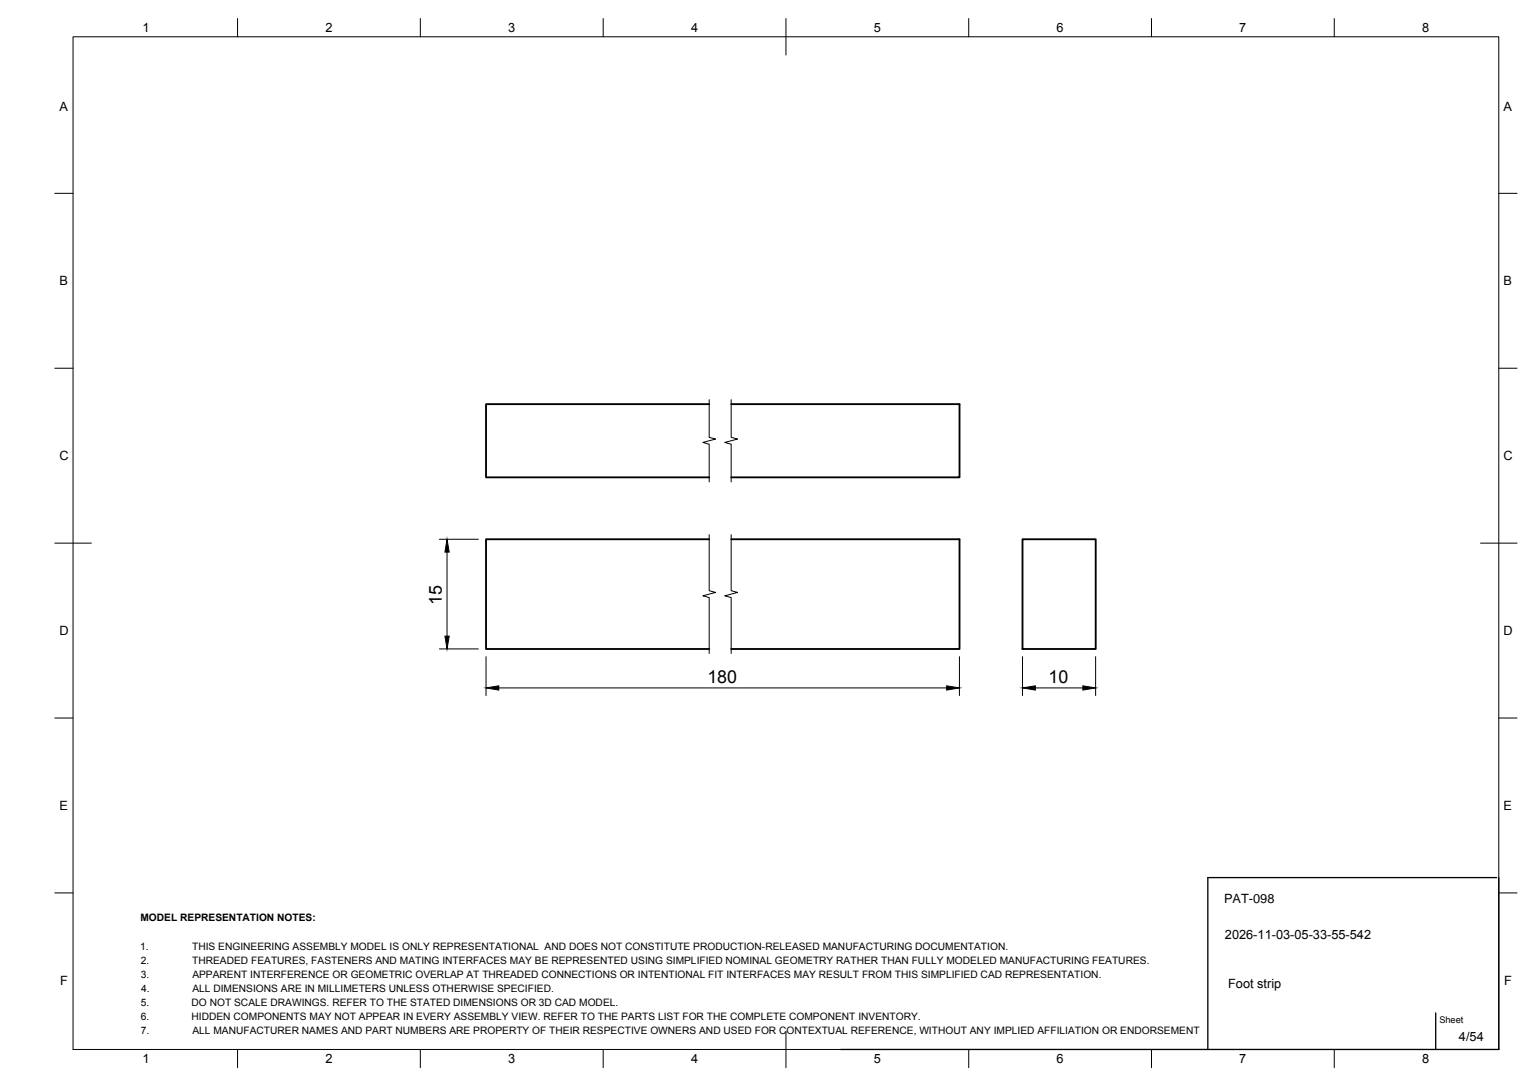
ISO-10303-21;
HEADER;
/* Generated by software containing ST-Developer
 * from STEP Tools, Inc. (www.steptools.com) 
 */

FILE_DESCRIPTION(
/* description */ ('Spring compression tester'),
/* implementation_level */ '2;1');

FILE_NAME(
/* name */ 'Foot strip.step',
/* time_stamp */ '2026-10-28T03:24:11-07:00',
/* author */ (''),
/* organization */ (''),
/* preprocessor_version */ 'ST-DEVELOPER v20.2',
/* originating_system */ 'Autodesk Translation Framework v15.17.0.0',
/* authorisation */ '');

FILE_SCHEMA (('AUTOMOTIVE_DESIGN { 1 0 10303 214 3 1 1 }'));
ENDSEC;

DATA;
#10=MECHANICAL_DESIGN_GEOMETRIC_PRESENTATION_REPRESENTATION('',(#1105),#43521);
#985=SHAPE_REPRESENTATION_RELATIONSHIP('SRR','None',#43797,#1045);
#1045=ADVANCED_BREP_SHAPE_REPRESENTATION('',(#1180),#43457);
#1105=STYLED_ITEM('',(#44188),#1180);
#1180=MANIFOLD_SOLID_BREP('Body1',#18542);
#1603=PLANE('',#19362);
#1604=PLANE('',#19363);
#1605=PLANE('',#19364);
#1606=PLANE('',#19365);
#1607=PLANE('',#19366);
#1608=PLANE('',#19367);
#2204=FACE_OUTER_BOUND('',#3287,.T.);
#2205=FACE_OUTER_BOUND('',#3288,.T.);
#2206=FACE_OUTER_BOUND('',#3289,.T.);
#2207=FACE_OUTER_BOUND('',#3290,.T.);
#2208=FACE_OUTER_BOUND('',#3291,.T.);
#2209=FACE_OUTER_BOUND('',#3292,.T.);
#3287=EDGE_LOOP('',(#12385,#12386,#12387,#12388));
#3288=EDGE_LOOP('',(#12389,#12390,#12391,#12392));
#3289=EDGE_LOOP('',(#12393,#12394,#12395,#12396));
#3290=EDGE_LOOP('',(#12397,#12398,#12399,#12400));
#3291=EDGE_LOOP('',(#12401,#12402,#12403,#12404));
#3292=EDGE_LOOP('',(#12405,#12406,#12407,#12408));
#4650=LINE('',#26633,#6082);
#4651=LINE('',#26635,#6083);
#4652=LINE('',#26637,#6084);
#4653=LINE('',#26638,#6085);
#4654=LINE('',#26641,#6086);
#4655=LINE('',#26643,#6087);
#4656=LINE('',#26644,#6088);
#4657=LINE('',#26647,#6089);
#4658=LINE('',#26649,#6090);
#4659=LINE('',#26650,#6091);
#4660=LINE('',#26652,#6092);
#4661=LINE('',#26653,#6093);
#6082=VECTOR('',#21398,1.);
#6083=VECTOR('',#21399,1.);
#6084=VECTOR('',#21400,1.);
#6085=VECTOR('',#21401,1.);
#6086=VECTOR('',#21404,1.);
#6087=VECTOR('',#21405,1.);
#6088=VECTOR('',#21406,1.);
#6089=VECTOR('',#21409,1.);
#6090=VECTOR('',#21410,1.);
#6091=VECTOR('',#21411,1.);
#6092=VECTOR('',#21414,1.);
#6093=VECTOR('',#21415,1.);
#8192=VERTEX_POINT('',#26631);
#8193=VERTEX_POINT('',#26632);
#8194=VERTEX_POINT('',#26634);
#8195=VERTEX_POINT('',#26636);
#8196=VERTEX_POINT('',#26640);
#8197=VERTEX_POINT('',#26642);
#8198=VERTEX_POINT('',#26646);
#8199=VERTEX_POINT('',#26648);
#9857=EDGE_CURVE('',#8192,#8193,#4650,.T.);
#9858=EDGE_CURVE('',#8193,#8194,#4651,.T.);
#9859=EDGE_CURVE('',#8195,#8194,#4652,.T.);
#9860=EDGE_CURVE('',#8192,#8195,#4653,.T.);
#9861=EDGE_CURVE('',#8196,#8192,#4654,.T.);
#9862=EDGE_CURVE('',#8197,#8195,#4655,.T.);
#9863=EDGE_CURVE('',#8196,#8197,#4656,.T.);
#9864=EDGE_CURVE('',#8198,#8196,#4657,.T.);
#9865=EDGE_CURVE('',#8199,#8197,#4658,.T.);
#9866=EDGE_CURVE('',#8198,#8199,#4659,.T.);
#9867=EDGE_CURVE('',#8193,#8198,#4660,.T.);
#9868=EDGE_CURVE('',#8194,#8199,#4661,.T.);
#12385=ORIENTED_EDGE('',*,*,#9857,.T.);
#12386=ORIENTED_EDGE('',*,*,#9858,.T.);
#12387=ORIENTED_EDGE('',*,*,#9859,.F.);
#12388=ORIENTED_EDGE('',*,*,#9860,.F.);
#12389=ORIENTED_EDGE('',*,*,#9861,.T.);
#12390=ORIENTED_EDGE('',*,*,#9860,.T.);
#12391=ORIENTED_EDGE('',*,*,#9862,.F.);
#12392=ORIENTED_EDGE('',*,*,#9863,.F.);
#12393=ORIENTED_EDGE('',*,*,#9864,.T.);
#12394=ORIENTED_EDGE('',*,*,#9863,.T.);
#12395=ORIENTED_EDGE('',*,*,#9865,.F.);
#12396=ORIENTED_EDGE('',*,*,#9866,.F.);
#12397=ORIENTED_EDGE('',*,*,#9867,.T.);
#12398=ORIENTED_EDGE('',*,*,#9866,.T.);
#12399=ORIENTED_EDGE('',*,*,#9868,.F.);
#12400=ORIENTED_EDGE('',*,*,#9858,.F.);
#12401=ORIENTED_EDGE('',*,*,#9868,.T.);
#12402=ORIENTED_EDGE('',*,*,#9865,.T.);
#12403=ORIENTED_EDGE('',*,*,#9862,.T.);
#12404=ORIENTED_EDGE('',*,*,#9859,.T.);
#12405=ORIENTED_EDGE('',*,*,#9867,.F.);
#12406=ORIENTED_EDGE('',*,*,#9857,.F.);
#12407=ORIENTED_EDGE('',*,*,#9861,.F.);
#12408=ORIENTED_EDGE('',*,*,#9864,.F.);
#17528=ADVANCED_FACE('',(#2204),#1603,.T.);
#17529=ADVANCED_FACE('',(#2205),#1604,.T.);
#17530=ADVANCED_FACE('',(#2206),#1605,.T.);
#17531=ADVANCED_FACE('',(#2207),#1606,.T.);
#17532=ADVANCED_FACE('',(#2208),#1607,.T.);
#17533=ADVANCED_FACE('',(#2209),#1608,.F.);
#18542=CLOSED_SHELL('',(#17528,#17529,#17530,#17531,#17532,#17533));
#19361=AXIS2_PLACEMENT_3D('',#26629,#21394,#21395);
#19362=AXIS2_PLACEMENT_3D('',#26630,#21396,#21397);
#19363=AXIS2_PLACEMENT_3D('',#26639,#21402,#21403);
#19364=AXIS2_PLACEMENT_3D('',#26645,#21407,#21408);
#19365=AXIS2_PLACEMENT_3D('',#26651,#21412,#21413);
#19366=AXIS2_PLACEMENT_3D('',#26654,#21416,#21417);
#19367=AXIS2_PLACEMENT_3D('',#26655,#21418,#21419);
#21394=DIRECTION('axis',(0.,0.,1.));
#21395=DIRECTION('refdir',(1.,0.,0.));
#21396=DIRECTION('center_axis',(0.,1.,0.));
#21397=DIRECTION('ref_axis',(-1.,0.,0.));
#21398=DIRECTION('',(-1.,0.,0.));
#21399=DIRECTION('',(0.,0.,1.));
#21400=DIRECTION('',(-1.,0.,0.));
#21401=DIRECTION('',(0.,0.,1.));
#21402=DIRECTION('center_axis',(1.,0.,0.));
#21403=DIRECTION('ref_axis',(0.,1.,0.));
#21404=DIRECTION('',(0.,1.,0.));
#21405=DIRECTION('',(0.,1.,0.));
#21406=DIRECTION('',(0.,0.,1.));
#21407=DIRECTION('center_axis',(0.,-1.,0.));
#21408=DIRECTION('ref_axis',(1.,0.,0.));
#21409=DIRECTION('',(1.,0.,0.));
#21410=DIRECTION('',(1.,0.,0.));
#21411=DIRECTION('',(0.,0.,1.));
#21412=DIRECTION('center_axis',(-1.,0.,0.));
#21413=DIRECTION('ref_axis',(0.,-1.,0.));
#21414=DIRECTION('',(0.,-1.,0.));
#21415=DIRECTION('',(0.,-1.,0.));
#21416=DIRECTION('center_axis',(0.,0.,1.));
#21417=DIRECTION('ref_axis',(1.,0.,0.));
#21418=DIRECTION('center_axis',(0.,0.,1.));
#21419=DIRECTION('ref_axis',(1.,0.,0.));
#26629=CARTESIAN_POINT('',(0.,0.,0.));
#26630=CARTESIAN_POINT('Origin',(9.,-3.,-2.2));
#26631=CARTESIAN_POINT('',(9.,-3.,-2.2));
#26632=CARTESIAN_POINT('',(-9.,-3.,-2.2));
#26633=CARTESIAN_POINT('',(9.,-3.,-2.2));
#26634=CARTESIAN_POINT('',(-9.,-3.,-1.2));
#26635=CARTESIAN_POINT('',(-9.,-3.,-2.2));
#26636=CARTESIAN_POINT('',(9.,-3.,-1.2));
#26637=CARTESIAN_POINT('',(9.,-3.,-1.2));
#26638=CARTESIAN_POINT('',(9.,-3.,-2.2));
#26639=CARTESIAN_POINT('Origin',(9.,-4.5,-2.2));
#26640=CARTESIAN_POINT('',(9.,-4.5,-2.2));
#26641=CARTESIAN_POINT('',(9.,-4.5,-2.2));
#26642=CARTESIAN_POINT('',(9.,-4.5,-1.2));
#26643=CARTESIAN_POINT('',(9.,-4.5,-1.2));
#26644=CARTESIAN_POINT('',(9.,-4.5,-2.2));
#26645=CARTESIAN_POINT('Origin',(-9.,-4.5,-2.2));
#26646=CARTESIAN_POINT('',(-9.,-4.5,-2.2));
#26647=CARTESIAN_POINT('',(-9.,-4.5,-2.2));
#26648=CARTESIAN_POINT('',(-9.,-4.5,-1.2));
#26649=CARTESIAN_POINT('',(-9.,-4.5,-1.2));
#26650=CARTESIAN_POINT('',(-9.,-4.5,-2.2));
#26651=CARTESIAN_POINT('Origin',(-9.,-3.,-2.2));
#26652=CARTESIAN_POINT('',(-9.,-3.,-2.2));
#26653=CARTESIAN_POINT('',(-9.,-3.,-1.2));
#26654=CARTESIAN_POINT('Origin',(0.,-3.75,-1.2));
#26655=CARTESIAN_POINT('Origin',(0.,-3.75,-2.2));
#43389=UNCERTAINTY_MEASURE_WITH_UNIT(LENGTH_MEASURE(0.001),#43522,
'DISTANCE_ACCURACY_VALUE',
'Maximum model space distance between geometric entities at asserted c
onnectivities');
#43453=UNCERTAINTY_MEASURE_WITH_UNIT(LENGTH_MEASURE(0.001),#43522,
'DISTANCE_ACCURACY_VALUE',
'Maximum model space distance between geometric entities at asserted c
onnectivities');
#43457=(
GEOMETRIC_REPRESENTATION_CONTEXT(3)
GLOBAL_UNCERTAINTY_ASSIGNED_CONTEXT((#43389))
GLOBAL_UNIT_ASSIGNED_CONTEXT((#43522,#43524,#43525))
REPRESENTATION_CONTEXT('','3D')
);
#43521=(
GEOMETRIC_REPRESENTATION_CONTEXT(3)
GLOBAL_UNCERTAINTY_ASSIGNED_CONTEXT((#43453))
GLOBAL_UNIT_ASSIGNED_CONTEXT((#43522,#43524,#43525))
REPRESENTATION_CONTEXT('','3D')
);
#43522=(
LENGTH_UNIT()
NAMED_UNIT(*)
SI_UNIT(.CENTI.,.METRE.)
);
#43524=(
NAMED_UNIT(*)
PLANE_ANGLE_UNIT()
SI_UNIT($,.RADIAN.)
);
#43525=(
NAMED_UNIT(*)
SI_UNIT($,.STERADIAN.)
SOLID_ANGLE_UNIT()
);
#43529=SHAPE_DEFINITION_REPRESENTATION(#43596,#43797);
#43596=PRODUCT_DEFINITION_SHAPE('',$,#43865);
#43797=SHAPE_REPRESENTATION('',(#19361),#43457);
#43861=PRODUCT_DEFINITION_CONTEXT('part definition',#44064,'design');
#43865=PRODUCT_DEFINITION('Foot strip','Foot strip',#43932,#43861);
#43932=PRODUCT_DEFINITION_FORMATION('',$,#44069);
#44064=APPLICATION_CONTEXT(
'Core Data for Automotive Mechanical Design Process');
#44065=PRODUCT_CONTEXT('part definition',#44064,'mechanical');
#44069=PRODUCT('Foot strip','Foot strip','Foot strip',(#44065));
#44182=COLOUR_RGB('Light Blue',0.38,0.62,0.78);
#44183=FILL_AREA_STYLE_COLOUR('',#44182);
#44184=FILL_AREA_STYLE('',(#44183));
#44185=SURFACE_STYLE_FILL_AREA(#44184);
#44186=SURFACE_SIDE_STYLE('',(#44185));
#44187=SURFACE_STYLE_USAGE(.BOTH.,#44186);
#44188=PRESENTATION_STYLE_ASSIGNMENT((#44187));
ENDSEC;
END-ISO-10303-21;
